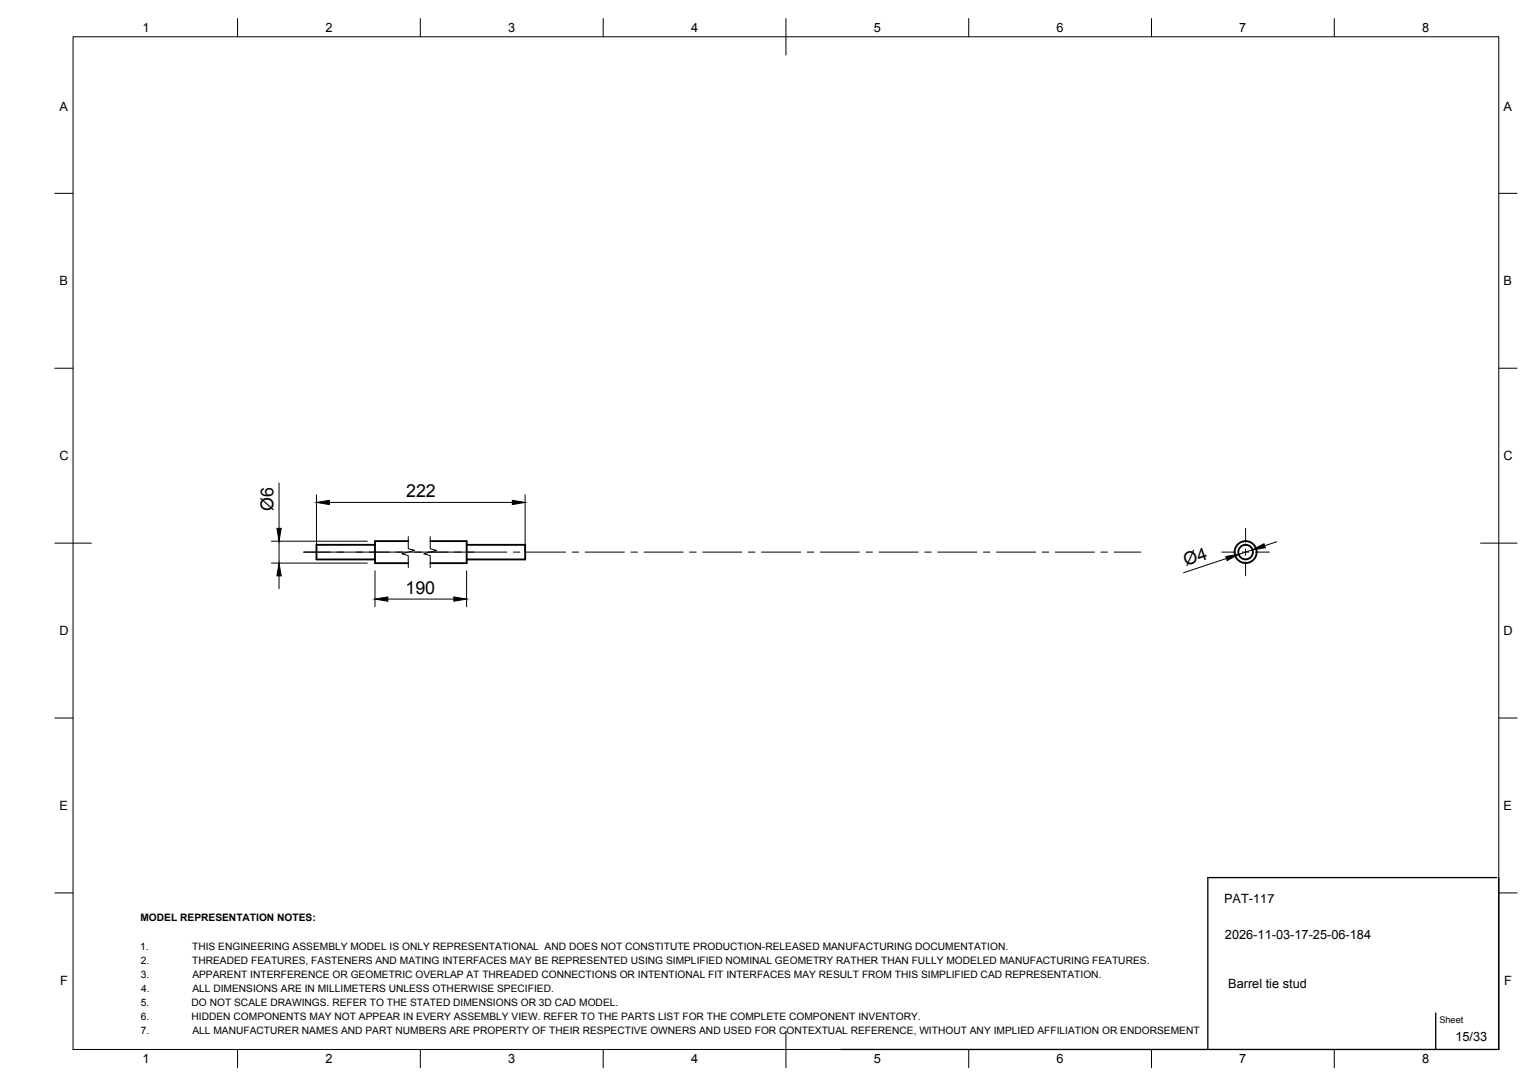
ISO-10303-21;
HEADER;
/* Generated by software containing ST-Developer
 * from STEP Tools, Inc. (www.steptools.com) 
 */

FILE_DESCRIPTION(
/* description */ ('Counterbalanced vertical column'),
/* implementation_level */ '2;1');

FILE_NAME(
/* name */ 'Barrel tie stud.step',
/* time_stamp */ '2026-10-29T16:47:22-07:00',
/* author */ (''),
/* organization */ (''),
/* preprocessor_version */ 'ST-DEVELOPER v20.2',
/* originating_system */ 'Autodesk Translation Framework v15.17.0.0',
/* authorisation */ '');

FILE_SCHEMA (('AUTOMOTIVE_DESIGN { 1 0 10303 214 3 1 1 }'));
ENDSEC;

DATA;
#10=MECHANICAL_DESIGN_GEOMETRIC_PRESENTATION_REPRESENTATION('',(#360),#15040);
#290=SHAPE_REPRESENTATION_RELATIONSHIP('SRR','None',#15194,#325);
#325=ADVANCED_BREP_SHAPE_REPRESENTATION('',(#395),#15013);
#360=STYLED_ITEM('',(#15464),#395);
#395=MANIFOLD_SOLID_BREP('Body1',#7083);
#460=FACE_BOUND('',#1365,.T.);
#461=FACE_BOUND('',#1367,.T.);
#591=PLANE('',#7658);
#592=PLANE('',#7661);
#593=PLANE('',#7669);
#594=PLANE('',#7670);
#915=FACE_OUTER_BOUND('',#1364,.T.);
#916=FACE_OUTER_BOUND('',#1366,.T.);
#917=FACE_OUTER_BOUND('',#1368,.T.);
#918=FACE_OUTER_BOUND('',#1369,.T.);
#919=FACE_OUTER_BOUND('',#1370,.T.);
#920=FACE_OUTER_BOUND('',#1371,.T.);
#921=FACE_OUTER_BOUND('',#1372,.T.);
#1364=EDGE_LOOP('',(#5154));
#1365=EDGE_LOOP('',(#5155));
#1366=EDGE_LOOP('',(#5156));
#1367=EDGE_LOOP('',(#5157));
#1368=EDGE_LOOP('',(#5158,#5159,#5160,#5161));
#1369=EDGE_LOOP('',(#5162,#5163,#5164,#5165));
#1370=EDGE_LOOP('',(#5166,#5167,#5168,#5169));
#1371=EDGE_LOOP('',(#5170));
#1372=EDGE_LOOP('',(#5171));
#1876=LINE('',#10756,#2547);
#1877=LINE('',#10759,#2548);
#1878=LINE('',#10764,#2549);
#2547=VECTOR('',#8680,0.300000000000001);
#2548=VECTOR('',#8683,0.199999999999999);
#2549=VECTOR('',#8690,0.199999999999999);
#3151=CIRCLE('',#7659,0.300000000000001);
#3152=CIRCLE('',#7660,0.199999999999999);
#3153=CIRCLE('',#7662,0.300000000000001);
#3154=CIRCLE('',#7663,0.199999999999999);
#3155=CIRCLE('',#7666,0.199999999999999);
#3156=CIRCLE('',#7668,0.199999999999999);
#3428=VERTEX_POINT('',#10746);
#3429=VERTEX_POINT('',#10748);
#3430=VERTEX_POINT('',#10751);
#3431=VERTEX_POINT('',#10753);
#3432=VERTEX_POINT('',#10758);
#3433=VERTEX_POINT('',#10762);
#4078=EDGE_CURVE('',#3428,#3428,#3151,.T.);
#4079=EDGE_CURVE('',#3429,#3429,#3152,.T.);
#4080=EDGE_CURVE('',#3430,#3430,#3153,.T.);
#4081=EDGE_CURVE('',#3431,#3431,#3154,.T.);
#4082=EDGE_CURVE('',#3428,#3430,#1876,.T.);
#4083=EDGE_CURVE('',#3431,#3432,#1877,.T.);
#4084=EDGE_CURVE('',#3432,#3432,#3155,.T.);
#4085=EDGE_CURVE('',#3433,#3433,#3156,.T.);
#4086=EDGE_CURVE('',#3433,#3429,#1878,.T.);
#5154=ORIENTED_EDGE('',*,*,#4078,.T.);
#5155=ORIENTED_EDGE('',*,*,#4079,.F.);
#5156=ORIENTED_EDGE('',*,*,#4080,.F.);
#5157=ORIENTED_EDGE('',*,*,#4081,.F.);
#5158=ORIENTED_EDGE('',*,*,#4078,.F.);
#5159=ORIENTED_EDGE('',*,*,#4082,.T.);
#5160=ORIENTED_EDGE('',*,*,#4080,.T.);
#5161=ORIENTED_EDGE('',*,*,#4082,.F.);
#5162=ORIENTED_EDGE('',*,*,#4081,.T.);
#5163=ORIENTED_EDGE('',*,*,#4083,.T.);
#5164=ORIENTED_EDGE('',*,*,#4084,.T.);
#5165=ORIENTED_EDGE('',*,*,#4083,.F.);
#5166=ORIENTED_EDGE('',*,*,#4085,.F.);
#5167=ORIENTED_EDGE('',*,*,#4086,.T.);
#5168=ORIENTED_EDGE('',*,*,#4079,.T.);
#5169=ORIENTED_EDGE('',*,*,#4086,.F.);
#5170=ORIENTED_EDGE('',*,*,#4085,.T.);
#5171=ORIENTED_EDGE('',*,*,#4084,.F.);
#6603=CYLINDRICAL_SURFACE('',#7664,0.300000000000001);
#6604=CYLINDRICAL_SURFACE('',#7665,0.199999999999999);
#6605=CYLINDRICAL_SURFACE('',#7667,0.199999999999999);
#6757=ADVANCED_FACE('',(#915,#460),#591,.T.);
#6758=ADVANCED_FACE('',(#916,#461),#592,.F.);
#6759=ADVANCED_FACE('',(#917),#6603,.T.);
#6760=ADVANCED_FACE('',(#918),#6604,.T.);
#6761=ADVANCED_FACE('',(#919),#6605,.T.);
#6762=ADVANCED_FACE('',(#920),#593,.T.);
#6763=ADVANCED_FACE('',(#921),#594,.F.);
#7083=CLOSED_SHELL('',(#6757,#6758,#6759,#6760,#6761,#6762,#6763));
#7657=AXIS2_PLACEMENT_3D('',#10744,#8664,#8665);
#7658=AXIS2_PLACEMENT_3D('',#10745,#8666,#8667);
#7659=AXIS2_PLACEMENT_3D('',#10747,#8668,#8669);
#7660=AXIS2_PLACEMENT_3D('',#10749,#8670,#8671);
#7661=AXIS2_PLACEMENT_3D('',#10750,#8672,#8673);
#7662=AXIS2_PLACEMENT_3D('',#10752,#8674,#8675);
#7663=AXIS2_PLACEMENT_3D('',#10754,#8676,#8677);
#7664=AXIS2_PLACEMENT_3D('',#10755,#8678,#8679);
#7665=AXIS2_PLACEMENT_3D('',#10757,#8681,#8682);
#7666=AXIS2_PLACEMENT_3D('',#10760,#8684,#8685);
#7667=AXIS2_PLACEMENT_3D('',#10761,#8686,#8687);
#7668=AXIS2_PLACEMENT_3D('',#10763,#8688,#8689);
#7669=AXIS2_PLACEMENT_3D('',#10765,#8691,#8692);
#7670=AXIS2_PLACEMENT_3D('',#10766,#8693,#8694);
#8664=DIRECTION('axis',(0.,0.,1.));
#8665=DIRECTION('refdir',(1.,0.,0.));
#8666=DIRECTION('center_axis',(0.,0.,1.));
#8667=DIRECTION('ref_axis',(1.,0.,0.));
#8668=DIRECTION('center_axis',(0.,0.,1.));
#8669=DIRECTION('ref_axis',(1.,0.,0.));
#8670=DIRECTION('center_axis',(0.,0.,1.));
#8671=DIRECTION('ref_axis',(1.,0.,0.));
#8672=DIRECTION('center_axis',(0.,0.,1.));
#8673=DIRECTION('ref_axis',(1.,0.,0.));
#8674=DIRECTION('center_axis',(0.,0.,1.));
#8675=DIRECTION('ref_axis',(1.,0.,0.));
#8676=DIRECTION('center_axis',(0.,0.,-1.));
#8677=DIRECTION('ref_axis',(1.,0.,0.));
#8678=DIRECTION('center_axis',(0.,0.,1.));
#8679=DIRECTION('ref_axis',(1.,0.,0.));
#8680=DIRECTION('',(0.,0.,-1.));
#8681=DIRECTION('center_axis',(0.,0.,1.));
#8682=DIRECTION('ref_axis',(1.,0.,0.));
#8683=DIRECTION('',(0.,0.,-1.));
#8684=DIRECTION('center_axis',(0.,0.,1.));
#8685=DIRECTION('ref_axis',(1.,0.,0.));
#8686=DIRECTION('center_axis',(0.,0.,1.));
#8687=DIRECTION('ref_axis',(1.,0.,0.));
#8688=DIRECTION('center_axis',(0.,0.,1.));
#8689=DIRECTION('ref_axis',(1.,0.,0.));
#8690=DIRECTION('',(0.,0.,-1.));
#8691=DIRECTION('center_axis',(0.,0.,1.));
#8692=DIRECTION('ref_axis',(1.,0.,0.));
#8693=DIRECTION('center_axis',(0.,0.,1.));
#8694=DIRECTION('ref_axis',(1.,0.,0.));
#10744=CARTESIAN_POINT('',(0.,0.,0.));
#10745=CARTESIAN_POINT('Origin',(-8.8,0.,20.));
#10746=CARTESIAN_POINT('',(-9.1,-3.67394039744207E-17,20.));
#10747=CARTESIAN_POINT('Origin',(-8.8,0.,20.));
#10748=CARTESIAN_POINT('',(-9.,-2.4492935982947E-17,20.));
#10749=CARTESIAN_POINT('Origin',(-8.8,0.,20.));
#10750=CARTESIAN_POINT('Origin',(-8.8,0.,1.));
#10751=CARTESIAN_POINT('',(-9.1,-3.67394039744207E-17,1.));
#10752=CARTESIAN_POINT('Origin',(-8.8,0.,1.));
#10753=CARTESIAN_POINT('',(-9.,2.4492935982947E-17,1.));
#10754=CARTESIAN_POINT('Origin',(-8.8,0.,1.));
#10755=CARTESIAN_POINT('Origin',(-8.8,0.,1.));
#10756=CARTESIAN_POINT('',(-9.1,-3.67394039744207E-17,1.));
#10757=CARTESIAN_POINT('Origin',(-8.8,0.,-0.6));
#10758=CARTESIAN_POINT('',(-9.,-2.4492935982947E-17,-0.6));
#10759=CARTESIAN_POINT('',(-9.,-2.4492935982947E-17,-0.6));
#10760=CARTESIAN_POINT('Origin',(-8.8,0.,-0.6));
#10761=CARTESIAN_POINT('Origin',(-8.8,0.,-0.6));
#10762=CARTESIAN_POINT('',(-9.,-2.4492935982947E-17,21.6));
#10763=CARTESIAN_POINT('Origin',(-8.8,0.,21.6));
#10764=CARTESIAN_POINT('',(-9.,-2.4492935982947E-17,-0.6));
#10765=CARTESIAN_POINT('Origin',(-8.8,0.,21.6));
#10766=CARTESIAN_POINT('Origin',(-8.8,0.,-0.6));
#14973=UNCERTAINTY_MEASURE_WITH_UNIT(LENGTH_MEASURE(0.001),#15041,
'DISTANCE_ACCURACY_VALUE',
'Maximum model space distance between geometric entities at asserted c
onnectivities');
#15000=UNCERTAINTY_MEASURE_WITH_UNIT(LENGTH_MEASURE(0.001),#15041,
'DISTANCE_ACCURACY_VALUE',
'Maximum model space distance between geometric entities at asserted c
onnectivities');
#15013=(
GEOMETRIC_REPRESENTATION_CONTEXT(3)
GLOBAL_UNCERTAINTY_ASSIGNED_CONTEXT((#14973))
GLOBAL_UNIT_ASSIGNED_CONTEXT((#15041,#15043,#15044))
REPRESENTATION_CONTEXT('','3D')
);
#15040=(
GEOMETRIC_REPRESENTATION_CONTEXT(3)
GLOBAL_UNCERTAINTY_ASSIGNED_CONTEXT((#15000))
GLOBAL_UNIT_ASSIGNED_CONTEXT((#15041,#15043,#15044))
REPRESENTATION_CONTEXT('','3D')
);
#15041=(
LENGTH_UNIT()
NAMED_UNIT(*)
SI_UNIT(.CENTI.,.METRE.)
);
#15043=(
NAMED_UNIT(*)
PLANE_ANGLE_UNIT()
SI_UNIT($,.RADIAN.)
);
#15044=(
NAMED_UNIT(*)
SI_UNIT($,.STERADIAN.)
SOLID_ANGLE_UNIT()
);
#15057=SHAPE_DEFINITION_REPRESENTATION(#15096,#15194);
#15096=PRODUCT_DEFINITION_SHAPE('',$,#15234);
#15194=SHAPE_REPRESENTATION('',(#7657),#15013);
#15221=PRODUCT_DEFINITION_CONTEXT('part definition',#15340,'design');
#15234=PRODUCT_DEFINITION('Barrel tie stud','Barrel tie stud',#15273,#15221);
#15273=PRODUCT_DEFINITION_FORMATION('',$,#15354);
#15340=APPLICATION_CONTEXT(
'Core Data for Automotive Mechanical Design Process');
#15341=PRODUCT_CONTEXT('part definition',#15340,'mechanical');
#15354=PRODUCT('Barrel tie stud','Barrel tie stud','Barrel tie stud',(#15341));
#15458=COLOUR_RGB('Black',0.12,0.14,0.17);
#15459=FILL_AREA_STYLE_COLOUR('',#15458);
#15460=FILL_AREA_STYLE('',(#15459));
#15461=SURFACE_STYLE_FILL_AREA(#15460);
#15462=SURFACE_SIDE_STYLE('',(#15461));
#15463=SURFACE_STYLE_USAGE(.BOTH.,#15462);
#15464=PRESENTATION_STYLE_ASSIGNMENT((#15463));
ENDSEC;
END-ISO-10303-21;
